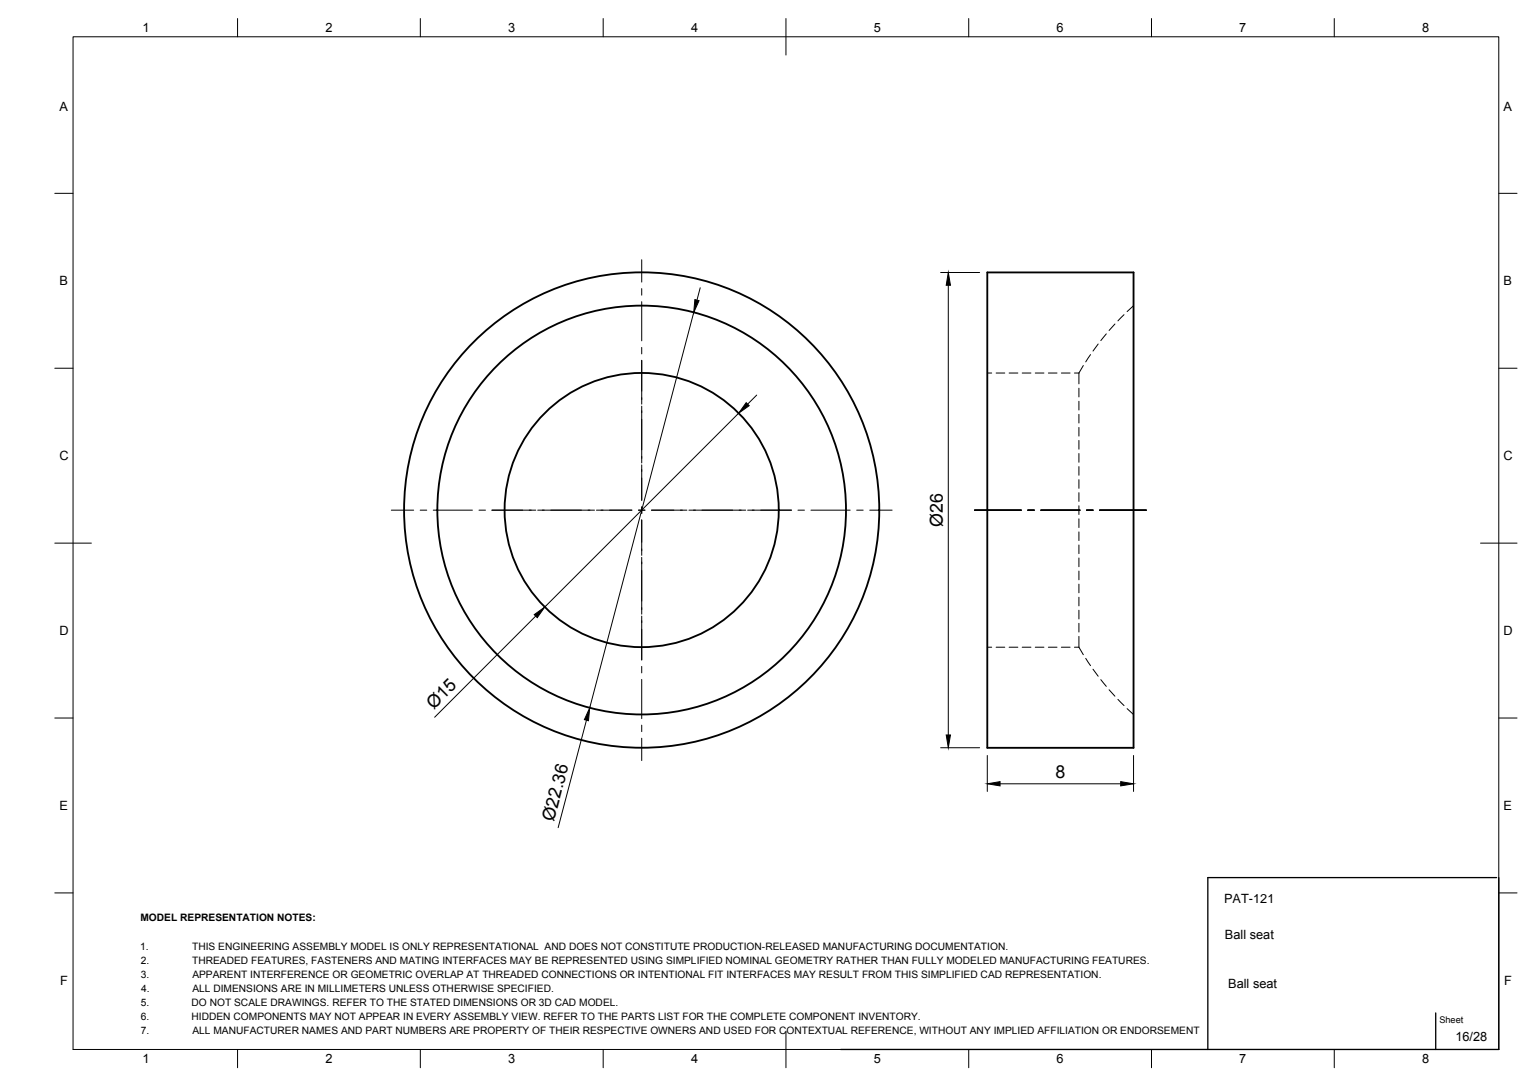
ISO-10303-21;
HEADER;
/* Generated by software containing ST-Developer
 * from STEP Tools, Inc. (www.steptools.com) 
 */

FILE_DESCRIPTION(
/* description */ ('Wall-mounted air drop station'),
/* implementation_level */ '2;1');

FILE_NAME(
/* name */ 'Ball seat.step',
/* time_stamp */ '2026-10-28T22:16:19-07:00',
/* author */ (''),
/* organization */ (''),
/* preprocessor_version */ 'ST-DEVELOPER v20.2',
/* originating_system */ 'Autodesk Translation Framework v15.17.0.0',
/* authorisation */ '');

FILE_SCHEMA (('AUTOMOTIVE_DESIGN { 1 0 10303 214 3 1 1 }'));
ENDSEC;

DATA;
#10=MECHANICAL_DESIGN_GEOMETRIC_PRESENTATION_REPRESENTATION('',(#356),#10517);
#260=SPHERICAL_SURFACE('',#6555,1.5);
#298=SHAPE_REPRESENTATION_RELATIONSHIP('SRR','None',#10655,#327);
#327=ADVANCED_BREP_SHAPE_REPRESENTATION('',(#385),#10499);
#356=STYLED_ITEM('',(#10860),#385);
#385=MANIFOLD_SOLID_BREP('Body1',#5895);
#489=FACE_BOUND('',#1370,.T.);
#490=FACE_BOUND('',#1374,.T.);
#491=FACE_BOUND('',#1376,.T.);
#627=PLANE('',#6563);
#628=PLANE('',#6564);
#924=FACE_OUTER_BOUND('',#1369,.T.);
#925=FACE_OUTER_BOUND('',#1371,.T.);
#926=FACE_OUTER_BOUND('',#1372,.T.);
#927=FACE_OUTER_BOUND('',#1373,.T.);
#928=FACE_OUTER_BOUND('',#1375,.T.);
#1369=EDGE_LOOP('',(#4697));
#1370=EDGE_LOOP('',(#4698));
#1371=EDGE_LOOP('',(#4699,#4700,#4701,#4702));
#1372=EDGE_LOOP('',(#4703,#4704,#4705,#4706));
#1373=EDGE_LOOP('',(#4707));
#1374=EDGE_LOOP('',(#4708));
#1375=EDGE_LOOP('',(#4709));
#1376=EDGE_LOOP('',(#4710));
#1818=LINE('',#9560,#2282);
#1819=LINE('',#9566,#2283);
#2282=VECTOR('',#7798,0.75);
#2283=VECTOR('',#7805,1.3);
#2656=CIRCLE('',#6556,1.11803398874989);
#2657=CIRCLE('',#6557,0.75);
#2658=CIRCLE('',#6559,0.75);
#2659=CIRCLE('',#6561,1.3);
#2660=CIRCLE('',#6562,1.3);
#3006=VERTEX_POINT('',#9554);
#3007=VERTEX_POINT('',#9556);
#3008=VERTEX_POINT('',#9559);
#3009=VERTEX_POINT('',#9563);
#3010=VERTEX_POINT('',#9565);
#3606=EDGE_CURVE('',#3006,#3006,#2656,.T.);
#3607=EDGE_CURVE('',#3007,#3007,#2657,.T.);
#3608=EDGE_CURVE('',#3007,#3008,#1818,.T.);
#3609=EDGE_CURVE('',#3008,#3008,#2658,.T.);
#3610=EDGE_CURVE('',#3009,#3009,#2659,.T.);
#3611=EDGE_CURVE('',#3009,#3010,#1819,.T.);
#3612=EDGE_CURVE('',#3010,#3010,#2660,.T.);
#4697=ORIENTED_EDGE('',*,*,#3606,.F.);
#4698=ORIENTED_EDGE('',*,*,#3607,.F.);
#4699=ORIENTED_EDGE('',*,*,#3607,.T.);
#4700=ORIENTED_EDGE('',*,*,#3608,.T.);
#4701=ORIENTED_EDGE('',*,*,#3609,.T.);
#4702=ORIENTED_EDGE('',*,*,#3608,.F.);
#4703=ORIENTED_EDGE('',*,*,#3610,.F.);
#4704=ORIENTED_EDGE('',*,*,#3611,.T.);
#4705=ORIENTED_EDGE('',*,*,#3612,.T.);
#4706=ORIENTED_EDGE('',*,*,#3611,.F.);
#4707=ORIENTED_EDGE('',*,*,#3610,.T.);
#4708=ORIENTED_EDGE('',*,*,#3606,.T.);
#4709=ORIENTED_EDGE('',*,*,#3612,.F.);
#4710=ORIENTED_EDGE('',*,*,#3609,.F.);
#5493=CYLINDRICAL_SURFACE('',#6558,0.75);
#5494=CYLINDRICAL_SURFACE('',#6560,1.3);
#5697=ADVANCED_FACE('',(#924,#489),#260,.F.);
#5698=ADVANCED_FACE('',(#925),#5493,.F.);
#5699=ADVANCED_FACE('',(#926),#5494,.T.);
#5700=ADVANCED_FACE('',(#927,#490),#627,.T.);
#5701=ADVANCED_FACE('',(#928,#491),#628,.F.);
#5895=CLOSED_SHELL('',(#5697,#5698,#5699,#5700,#5701));
#6554=AXIS2_PLACEMENT_3D('',#9552,#7788,#7789);
#6555=AXIS2_PLACEMENT_3D('',#9553,#7790,#7791);
#6556=AXIS2_PLACEMENT_3D('',#9555,#7792,#7793);
#6557=AXIS2_PLACEMENT_3D('',#9557,#7794,#7795);
#6558=AXIS2_PLACEMENT_3D('',#9558,#7796,#7797);
#6559=AXIS2_PLACEMENT_3D('',#9561,#7799,#7800);
#6560=AXIS2_PLACEMENT_3D('',#9562,#7801,#7802);
#6561=AXIS2_PLACEMENT_3D('',#9564,#7803,#7804);
#6562=AXIS2_PLACEMENT_3D('',#9567,#7806,#7807);
#6563=AXIS2_PLACEMENT_3D('',#9568,#7808,#7809);
#6564=AXIS2_PLACEMENT_3D('',#9569,#7810,#7811);
#7788=DIRECTION('axis',(0.,0.,1.));
#7789=DIRECTION('refdir',(1.,0.,0.));
#7790=DIRECTION('center_axis',(6.12323399573677E-17,0.,1.));
#7791=DIRECTION('ref_axis',(1.,0.,0.));
#7792=DIRECTION('center_axis',(0.,-1.,0.));
#7793=DIRECTION('ref_axis',(0.,0.,-1.));
#7794=DIRECTION('center_axis',(0.,1.,0.));
#7795=DIRECTION('ref_axis',(1.,0.,0.));
#7796=DIRECTION('center_axis',(0.,1.,0.));
#7797=DIRECTION('ref_axis',(1.,0.,0.));
#7798=DIRECTION('',(0.,-1.,0.));
#7799=DIRECTION('center_axis',(0.,-1.,0.));
#7800=DIRECTION('ref_axis',(1.,0.,0.));
#7801=DIRECTION('center_axis',(0.,1.,0.));
#7802=DIRECTION('ref_axis',(1.,0.,0.));
#7803=DIRECTION('center_axis',(0.,1.,0.));
#7804=DIRECTION('ref_axis',(1.,0.,0.));
#7805=DIRECTION('',(0.,-1.,0.));
#7806=DIRECTION('center_axis',(0.,1.,0.));
#7807=DIRECTION('ref_axis',(1.,0.,0.));
#7808=DIRECTION('center_axis',(0.,1.,0.));
#7809=DIRECTION('ref_axis',(1.,0.,0.));
#7810=DIRECTION('center_axis',(0.,1.,0.));
#7811=DIRECTION('ref_axis',(1.,0.,0.));
#9552=CARTESIAN_POINT('',(0.,0.,0.));
#9553=CARTESIAN_POINT('Origin',(0.,0.,5.));
#9554=CARTESIAN_POINT('',(-1.36919674566051E-16,-1.,6.11803398874989));
#9555=CARTESIAN_POINT('Origin',(0.,-1.,5.));
#9556=CARTESIAN_POINT('',(-0.75,-1.29903810567666,5.));
#9557=CARTESIAN_POINT('Origin',(0.,-1.29903810567666,5.));
#9558=CARTESIAN_POINT('Origin',(0.,-1.8,5.));
#9559=CARTESIAN_POINT('',(-0.75,-1.8,5.));
#9560=CARTESIAN_POINT('',(-0.75,-1.8,5.));
#9561=CARTESIAN_POINT('Origin',(0.,-1.8,5.));
#9562=CARTESIAN_POINT('Origin',(0.,-1.8,5.));
#9563=CARTESIAN_POINT('',(-1.3,-1.,5.));
#9564=CARTESIAN_POINT('Origin',(0.,-1.,5.));
#9565=CARTESIAN_POINT('',(-1.3,-1.8,5.));
#9566=CARTESIAN_POINT('',(-1.3,-1.8,5.));
#9567=CARTESIAN_POINT('Origin',(0.,-1.8,5.));
#9568=CARTESIAN_POINT('Origin',(0.,-1.,5.));
#9569=CARTESIAN_POINT('Origin',(0.,-1.8,5.));
#10466=UNCERTAINTY_MEASURE_WITH_UNIT(LENGTH_MEASURE(0.001),#10518,
'DISTANCE_ACCURACY_VALUE',
'Maximum model space distance between geometric entities at asserted c
onnectivities');
#10484=UNCERTAINTY_MEASURE_WITH_UNIT(LENGTH_MEASURE(0.001),#10518,
'DISTANCE_ACCURACY_VALUE',
'Maximum model space distance between geometric entities at asserted c
onnectivities');
#10499=(
GEOMETRIC_REPRESENTATION_CONTEXT(3)
GLOBAL_UNCERTAINTY_ASSIGNED_CONTEXT((#10466))
GLOBAL_UNIT_ASSIGNED_CONTEXT((#10518,#10520,#10521))
REPRESENTATION_CONTEXT('','3D')
);
#10517=(
GEOMETRIC_REPRESENTATION_CONTEXT(3)
GLOBAL_UNCERTAINTY_ASSIGNED_CONTEXT((#10484))
GLOBAL_UNIT_ASSIGNED_CONTEXT((#10518,#10520,#10521))
REPRESENTATION_CONTEXT('','3D')
);
#10518=(
LENGTH_UNIT()
NAMED_UNIT(*)
SI_UNIT(.CENTI.,.METRE.)
);
#10520=(
NAMED_UNIT(*)
PLANE_ANGLE_UNIT()
SI_UNIT($,.RADIAN.)
);
#10521=(
NAMED_UNIT(*)
SI_UNIT($,.STERADIAN.)
SOLID_ANGLE_UNIT()
);
#10536=SHAPE_DEFINITION_REPRESENTATION(#10568,#10655);
#10568=PRODUCT_DEFINITION_SHAPE('',$,#10688);
#10655=SHAPE_REPRESENTATION('',(#6554),#10499);
#10673=PRODUCT_DEFINITION_CONTEXT('part definition',#10771,'design');
#10688=PRODUCT_DEFINITION('Ball seat','Ball seat',#10720,#10673);
#10720=PRODUCT_DEFINITION_FORMATION('',$,#10787);
#10771=APPLICATION_CONTEXT(
'Core Data for Automotive Mechanical Design Process');
#10772=PRODUCT_CONTEXT('part definition',#10771,'mechanical');
#10787=PRODUCT('Ball seat','Ball seat','Ball seat',(#10772));
#10854=COLOUR_RGB('Light Blue',0.38,0.62,0.78);
#10855=FILL_AREA_STYLE_COLOUR('',#10854);
#10856=FILL_AREA_STYLE('',(#10855));
#10857=SURFACE_STYLE_FILL_AREA(#10856);
#10858=SURFACE_SIDE_STYLE('',(#10857));
#10859=SURFACE_STYLE_USAGE(.BOTH.,#10858);
#10860=PRESENTATION_STYLE_ASSIGNMENT((#10859));
ENDSEC;
END-ISO-10303-21;
